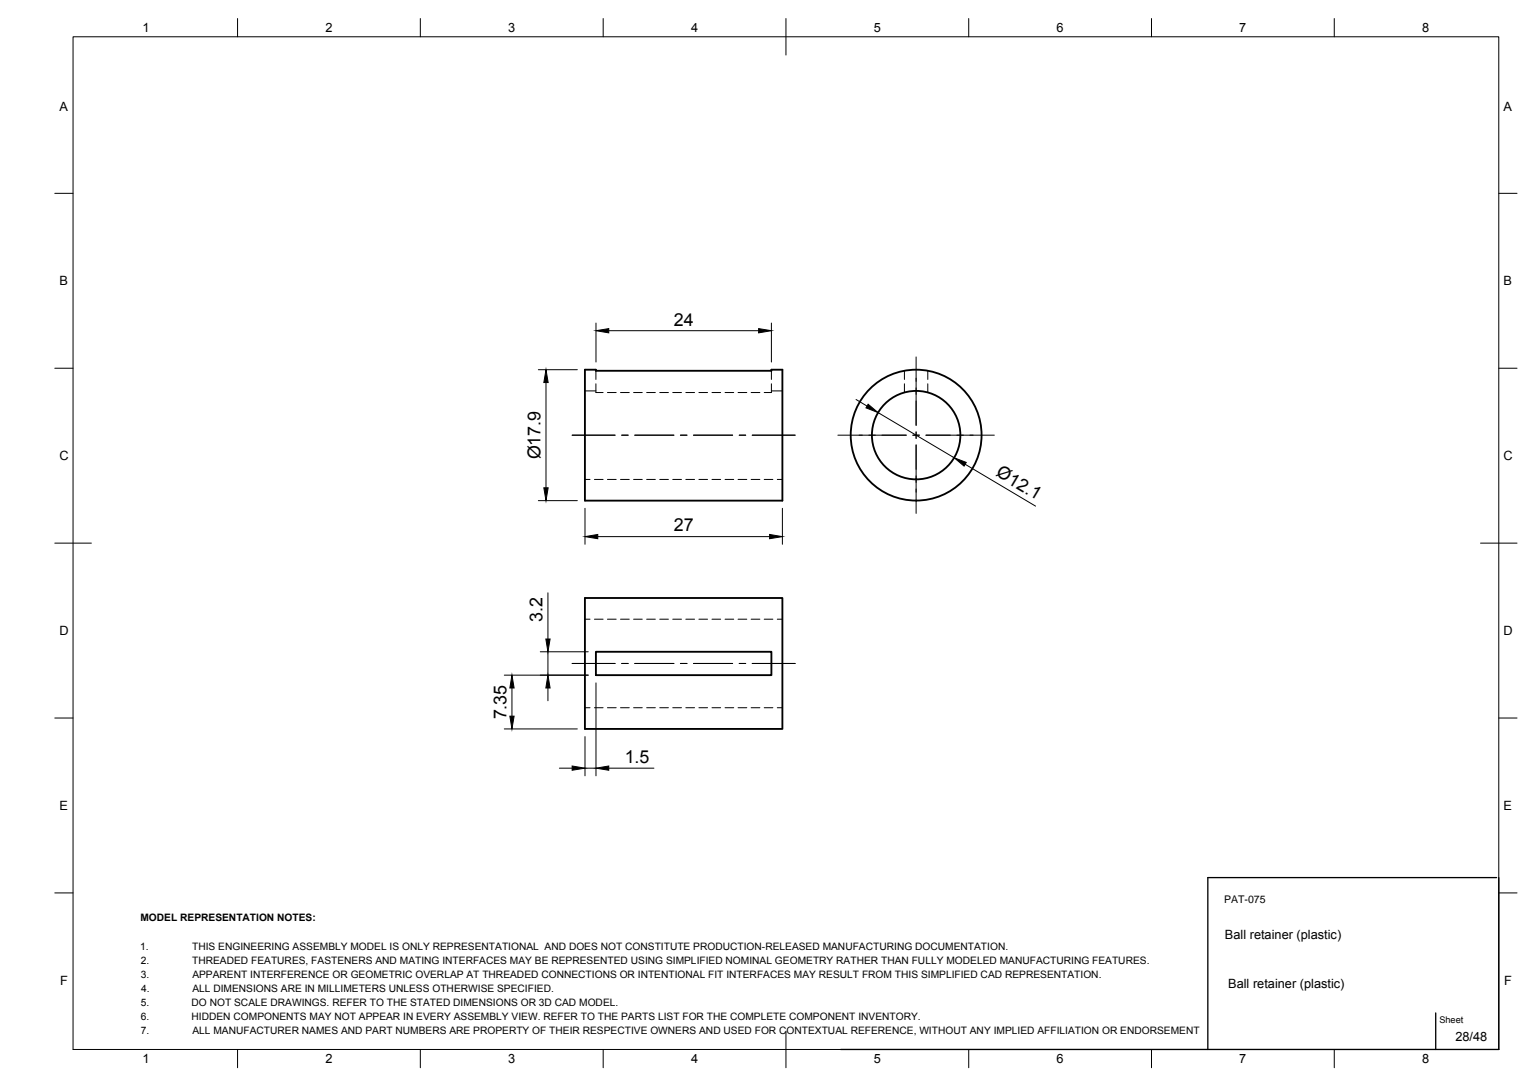
ISO-10303-21;
HEADER;
/* Generated by software containing ST-Developer
 * from STEP Tools, Inc. (www.steptools.com) 
 */

FILE_DESCRIPTION(
/* description */ ('Over-Centre Plunger Toggle Clamp on Slotted Fixture Frame'),
/* implementation_level */ '2;1');

FILE_NAME(
/* name */ 
'Ball retainer (plastic).step',
/* time_stamp */ '2026-10-28T03:23:24-07:00',
/* author */ (''),
/* organization */ (''),
/* preprocessor_version */ 'ST-DEVELOPER v20.2',
/* originating_system */ 'Autodesk Translation Framework v15.17.0.0',
/* authorisation */ '');

FILE_SCHEMA (('AUTOMOTIVE_DESIGN { 1 0 10303 214 3 1 1 }'));
ENDSEC;

DATA;
#10=MECHANICAL_DESIGN_GEOMETRIC_PRESENTATION_REPRESENTATION('',(#543),#15212);
#451=SHAPE_REPRESENTATION_RELATIONSHIP('SRR','None',#15427,#493);
#493=ADVANCED_BREP_SHAPE_REPRESENTATION('',(#593),#15189);
#543=STYLED_ITEM('',(#15712),#593);
#593=MANIFOLD_SOLID_BREP('Body1',#8276);
#736=FACE_BOUND('',#2002,.T.);
#737=FACE_BOUND('',#2004,.T.);
#738=FACE_BOUND('',#2006,.T.);
#739=FACE_BOUND('',#2008,.T.);
#966=PLANE('',#9332);
#967=PLANE('',#9335);
#968=PLANE('',#9336);
#969=PLANE('',#9339);
#970=PLANE('',#9340);
#971=PLANE('',#9345);
#1386=FACE_OUTER_BOUND('',#1997,.T.);
#1387=FACE_OUTER_BOUND('',#1998,.T.);
#1388=FACE_OUTER_BOUND('',#1999,.T.);
#1389=FACE_OUTER_BOUND('',#2000,.T.);
#1390=FACE_OUTER_BOUND('',#2001,.T.);
#1391=FACE_OUTER_BOUND('',#2003,.T.);
#1392=FACE_OUTER_BOUND('',#2005,.T.);
#1393=FACE_OUTER_BOUND('',#2007,.T.);
#1997=EDGE_LOOP('',(#6901,#6902,#6903,#6904));
#1998=EDGE_LOOP('',(#6905,#6906,#6907,#6908));
#1999=EDGE_LOOP('',(#6909,#6910,#6911,#6912));
#2000=EDGE_LOOP('',(#6913,#6914,#6915,#6916));
#2001=EDGE_LOOP('',(#6917));
#2002=EDGE_LOOP('',(#6918));
#2003=EDGE_LOOP('',(#6919,#6920,#6921,#6922));
#2004=EDGE_LOOP('',(#6923,#6924,#6925,#6926));
#2005=EDGE_LOOP('',(#6927));
#2006=EDGE_LOOP('',(#6928));
#2007=EDGE_LOOP('',(#6929,#6930,#6931,#6932));
#2008=EDGE_LOOP('',(#6933,#6934,#6935,#6936));
#2641=LINE('',#14158,#3271);
#2642=LINE('',#14161,#3272);
#2643=LINE('',#14164,#3273);
#2644=LINE('',#14166,#3274);
#2645=LINE('',#14167,#3275);
#2646=LINE('',#14173,#3276);
#2647=LINE('',#14175,#3277);
#2648=LINE('',#14176,#3278);
#2649=LINE('',#14185,#3279);
#2650=LINE('',#14190,#3280);
#3271=VECTOR('',#11306,1.);
#3272=VECTOR('',#11309,1.);
#3273=VECTOR('',#11312,1.);
#3274=VECTOR('',#11313,1.);
#3275=VECTOR('',#11314,1.);
#3276=VECTOR('',#11321,1.);
#3277=VECTOR('',#11324,1.);
#3278=VECTOR('',#11325,1.);
#3279=VECTOR('',#11336,0.895);
#3280=VECTOR('',#11343,0.605);
#3727=CIRCLE('',#9333,0.895);
#3728=CIRCLE('',#9334,0.605);
#3729=CIRCLE('',#9337,0.895);
#3730=CIRCLE('',#9338,0.605);
#3731=CIRCLE('',#9341,0.895);
#3732=CIRCLE('',#9342,0.605);
#3733=CIRCLE('',#9344,0.895);
#3734=CIRCLE('',#9346,0.605);
#4311=VERTEX_POINT('',#14154);
#4312=VERTEX_POINT('',#14155);
#4313=VERTEX_POINT('',#14157);
#4314=VERTEX_POINT('',#14159);
#4315=VERTEX_POINT('',#14163);
#4316=VERTEX_POINT('',#14165);
#4317=VERTEX_POINT('',#14169);
#4318=VERTEX_POINT('',#14171);
#4319=VERTEX_POINT('',#14178);
#4320=VERTEX_POINT('',#14180);
#4321=VERTEX_POINT('',#14183);
#4322=VERTEX_POINT('',#14187);
#5211=EDGE_CURVE('',#4311,#4312,#3727,.T.);
#5212=EDGE_CURVE('',#4313,#4311,#2641,.T.);
#5213=EDGE_CURVE('',#4314,#4313,#3728,.T.);
#5214=EDGE_CURVE('',#4312,#4314,#2642,.T.);
#5215=EDGE_CURVE('',#4312,#4315,#2643,.T.);
#5216=EDGE_CURVE('',#4316,#4314,#2644,.T.);
#5217=EDGE_CURVE('',#4316,#4315,#2645,.T.);
#5218=EDGE_CURVE('',#4315,#4317,#3729,.T.);
#5219=EDGE_CURVE('',#4318,#4316,#3730,.T.);
#5220=EDGE_CURVE('',#4317,#4318,#2646,.T.);
#5221=EDGE_CURVE('',#4317,#4311,#2647,.T.);
#5222=EDGE_CURVE('',#4313,#4318,#2648,.T.);
#5223=EDGE_CURVE('',#4319,#4319,#3731,.T.);
#5224=EDGE_CURVE('',#4320,#4320,#3732,.T.);
#5225=EDGE_CURVE('',#4321,#4321,#3733,.T.);
#5226=EDGE_CURVE('',#4321,#4319,#2649,.T.);
#5227=EDGE_CURVE('',#4322,#4322,#3734,.T.);
#5228=EDGE_CURVE('',#4322,#4320,#2650,.T.);
#6901=ORIENTED_EDGE('',*,*,#5211,.F.);
#6902=ORIENTED_EDGE('',*,*,#5212,.F.);
#6903=ORIENTED_EDGE('',*,*,#5213,.F.);
#6904=ORIENTED_EDGE('',*,*,#5214,.F.);
#6905=ORIENTED_EDGE('',*,*,#5215,.F.);
#6906=ORIENTED_EDGE('',*,*,#5214,.T.);
#6907=ORIENTED_EDGE('',*,*,#5216,.F.);
#6908=ORIENTED_EDGE('',*,*,#5217,.T.);
#6909=ORIENTED_EDGE('',*,*,#5218,.F.);
#6910=ORIENTED_EDGE('',*,*,#5217,.F.);
#6911=ORIENTED_EDGE('',*,*,#5219,.F.);
#6912=ORIENTED_EDGE('',*,*,#5220,.F.);
#6913=ORIENTED_EDGE('',*,*,#5221,.F.);
#6914=ORIENTED_EDGE('',*,*,#5220,.T.);
#6915=ORIENTED_EDGE('',*,*,#5222,.F.);
#6916=ORIENTED_EDGE('',*,*,#5212,.T.);
#6917=ORIENTED_EDGE('',*,*,#5223,.F.);
#6918=ORIENTED_EDGE('',*,*,#5224,.T.);
#6919=ORIENTED_EDGE('',*,*,#5225,.F.);
#6920=ORIENTED_EDGE('',*,*,#5226,.T.);
#6921=ORIENTED_EDGE('',*,*,#5223,.T.);
#6922=ORIENTED_EDGE('',*,*,#5226,.F.);
#6923=ORIENTED_EDGE('',*,*,#5218,.T.);
#6924=ORIENTED_EDGE('',*,*,#5221,.T.);
#6925=ORIENTED_EDGE('',*,*,#5211,.T.);
#6926=ORIENTED_EDGE('',*,*,#5215,.T.);
#6927=ORIENTED_EDGE('',*,*,#5225,.T.);
#6928=ORIENTED_EDGE('',*,*,#5227,.F.);
#6929=ORIENTED_EDGE('',*,*,#5227,.T.);
#6930=ORIENTED_EDGE('',*,*,#5228,.T.);
#6931=ORIENTED_EDGE('',*,*,#5224,.F.);
#6932=ORIENTED_EDGE('',*,*,#5228,.F.);
#6933=ORIENTED_EDGE('',*,*,#5219,.T.);
#6934=ORIENTED_EDGE('',*,*,#5216,.T.);
#6935=ORIENTED_EDGE('',*,*,#5213,.T.);
#6936=ORIENTED_EDGE('',*,*,#5222,.T.);
#7707=CYLINDRICAL_SURFACE('',#9343,0.895);
#7708=CYLINDRICAL_SURFACE('',#9347,0.605);
#8058=ADVANCED_FACE('',(#1386),#966,.F.);
#8059=ADVANCED_FACE('',(#1387),#967,.F.);
#8060=ADVANCED_FACE('',(#1388),#968,.F.);
#8061=ADVANCED_FACE('',(#1389),#969,.F.);
#8062=ADVANCED_FACE('',(#1390,#736),#970,.T.);
#8063=ADVANCED_FACE('',(#1391,#737),#7707,.T.);
#8064=ADVANCED_FACE('',(#1392,#738),#971,.T.);
#8065=ADVANCED_FACE('',(#1393,#739),#7708,.F.);
#8276=CLOSED_SHELL('',(#8058,#8059,#8060,#8061,#8062,#8063,#8064,#8065));
#9331=AXIS2_PLACEMENT_3D('',#14152,#11300,#11301);
#9332=AXIS2_PLACEMENT_3D('',#14153,#11302,#11303);
#9333=AXIS2_PLACEMENT_3D('',#14156,#11304,#11305);
#9334=AXIS2_PLACEMENT_3D('',#14160,#11307,#11308);
#9335=AXIS2_PLACEMENT_3D('',#14162,#11310,#11311);
#9336=AXIS2_PLACEMENT_3D('',#14168,#11315,#11316);
#9337=AXIS2_PLACEMENT_3D('',#14170,#11317,#11318);
#9338=AXIS2_PLACEMENT_3D('',#14172,#11319,#11320);
#9339=AXIS2_PLACEMENT_3D('',#14174,#11322,#11323);
#9340=AXIS2_PLACEMENT_3D('',#14177,#11326,#11327);
#9341=AXIS2_PLACEMENT_3D('',#14179,#11328,#11329);
#9342=AXIS2_PLACEMENT_3D('',#14181,#11330,#11331);
#9343=AXIS2_PLACEMENT_3D('',#14182,#11332,#11333);
#9344=AXIS2_PLACEMENT_3D('',#14184,#11334,#11335);
#9345=AXIS2_PLACEMENT_3D('',#14186,#11337,#11338);
#9346=AXIS2_PLACEMENT_3D('',#14188,#11339,#11340);
#9347=AXIS2_PLACEMENT_3D('',#14189,#11341,#11342);
#11300=DIRECTION('axis',(0.,0.,1.));
#11301=DIRECTION('refdir',(1.,0.,0.));
#11302=DIRECTION('center_axis',(0.,1.,0.));
#11303=DIRECTION('ref_axis',(0.,0.,1.));
#11304=DIRECTION('center_axis',(0.,1.,0.));
#11305=DIRECTION('ref_axis',(1.,0.,0.));
#11306=DIRECTION('',(1.,0.,0.));
#11307=DIRECTION('center_axis',(0.,-1.,0.));
#11308=DIRECTION('ref_axis',(1.,0.,0.));
#11309=DIRECTION('',(-1.,0.,0.));
#11310=DIRECTION('center_axis',(0.,0.,-1.));
#11311=DIRECTION('ref_axis',(-1.,0.,0.));
#11312=DIRECTION('',(0.,-1.,0.));
#11313=DIRECTION('',(0.,1.,0.));
#11314=DIRECTION('',(1.,0.,0.));
#11315=DIRECTION('center_axis',(0.,-1.,0.));
#11316=DIRECTION('ref_axis',(0.,0.,-1.));
#11317=DIRECTION('center_axis',(0.,-1.,0.));
#11318=DIRECTION('ref_axis',(1.,0.,0.));
#11319=DIRECTION('center_axis',(0.,1.,0.));
#11320=DIRECTION('ref_axis',(1.,0.,0.));
#11321=DIRECTION('',(-1.,0.,0.));
#11322=DIRECTION('center_axis',(0.,0.,1.));
#11323=DIRECTION('ref_axis',(1.,0.,0.));
#11324=DIRECTION('',(0.,1.,0.));
#11325=DIRECTION('',(0.,-1.,0.));
#11326=DIRECTION('center_axis',(0.,1.,0.));
#11327=DIRECTION('ref_axis',(0.,0.,1.));
#11328=DIRECTION('center_axis',(0.,-1.,0.));
#11329=DIRECTION('ref_axis',(1.,0.,0.));
#11330=DIRECTION('center_axis',(0.,-1.,0.));
#11331=DIRECTION('ref_axis',(1.,0.,0.));
#11332=DIRECTION('center_axis',(0.,-1.,0.));
#11333=DIRECTION('ref_axis',(1.,0.,0.));
#11334=DIRECTION('center_axis',(0.,-1.,0.));
#11335=DIRECTION('ref_axis',(1.,0.,0.));
#11336=DIRECTION('',(0.,1.,0.));
#11337=DIRECTION('center_axis',(0.,-1.,0.));
#11338=DIRECTION('ref_axis',(0.,0.,-1.));
#11339=DIRECTION('center_axis',(0.,-1.,0.));
#11340=DIRECTION('ref_axis',(1.,0.,0.));
#11341=DIRECTION('center_axis',(0.,-1.,0.));
#11342=DIRECTION('ref_axis',(1.,0.,0.));
#11343=DIRECTION('',(0.,1.,0.));
#14152=CARTESIAN_POINT('',(0.,0.,0.));
#14153=CARTESIAN_POINT('Origin',(0.75,1.2,0.));
#14154=CARTESIAN_POINT('',(0.880582193778639,1.2,0.16));
#14155=CARTESIAN_POINT('',(0.880582193778639,1.2,-0.16));
#14156=CARTESIAN_POINT('Origin',(0.,1.2,0.));
#14157=CARTESIAN_POINT('',(0.583459510163302,1.2,0.16));
#14158=CARTESIAN_POINT('',(0.57,1.2,0.16));
#14159=CARTESIAN_POINT('',(0.583459510163302,1.2,-0.16));
#14160=CARTESIAN_POINT('Origin',(0.,1.2,0.));
#14161=CARTESIAN_POINT('',(0.93,1.2,-0.16));
#14162=CARTESIAN_POINT('Origin',(0.93,0.,-0.16));
#14163=CARTESIAN_POINT('',(0.880582193778639,-1.2,-0.16));
#14164=CARTESIAN_POINT('',(0.880582193778639,0.,-0.16));
#14165=CARTESIAN_POINT('',(0.583459510163302,-1.2,-0.16));
#14166=CARTESIAN_POINT('',(0.583459510163302,0.,-0.16));
#14167=CARTESIAN_POINT('',(0.93,-1.2,-0.16));
#14168=CARTESIAN_POINT('Origin',(0.75,-1.2,0.));
#14169=CARTESIAN_POINT('',(0.880582193778639,-1.2,0.16));
#14170=CARTESIAN_POINT('Origin',(0.,-1.2,0.));
#14171=CARTESIAN_POINT('',(0.583459510163302,-1.2,0.16));
#14172=CARTESIAN_POINT('Origin',(0.,-1.2,0.));
#14173=CARTESIAN_POINT('',(0.57,-1.2,0.16));
#14174=CARTESIAN_POINT('Origin',(0.57,0.,0.16));
#14175=CARTESIAN_POINT('',(0.880582193778639,0.,0.16));
#14176=CARTESIAN_POINT('',(0.583459510163302,0.,0.16));
#14177=CARTESIAN_POINT('Origin',(0.895,1.35,0.));
#14178=CARTESIAN_POINT('',(-0.895,1.35,-1.09605888523688E-16));
#14179=CARTESIAN_POINT('Origin',(0.,1.35,0.));
#14180=CARTESIAN_POINT('',(-0.605,1.35,-7.40911313484149E-17));
#14181=CARTESIAN_POINT('Origin',(0.,1.35,0.));
#14182=CARTESIAN_POINT('Origin',(0.,0.,0.));
#14183=CARTESIAN_POINT('',(-0.895,-1.35,-1.09605888523688E-16));
#14184=CARTESIAN_POINT('Origin',(0.,-1.35,0.));
#14185=CARTESIAN_POINT('',(-0.895,0.,-1.09605888523688E-16));
#14186=CARTESIAN_POINT('Origin',(0.605,-1.35,0.));
#14187=CARTESIAN_POINT('',(-0.605,-1.35,-7.40911313484149E-17));
#14188=CARTESIAN_POINT('Origin',(0.,-1.35,0.));
#14189=CARTESIAN_POINT('Origin',(0.,0.,0.));
#14190=CARTESIAN_POINT('',(-0.605,0.,-7.40911313484149E-17));
#15139=UNCERTAINTY_MEASURE_WITH_UNIT(LENGTH_MEASURE(0.001),#15213,
'DISTANCE_ACCURACY_VALUE',
'Maximum model space distance between geometric entities at asserted c
onnectivities');
#15162=UNCERTAINTY_MEASURE_WITH_UNIT(LENGTH_MEASURE(0.001),#15213,
'DISTANCE_ACCURACY_VALUE',
'Maximum model space distance between geometric entities at asserted c
onnectivities');
#15189=(
GEOMETRIC_REPRESENTATION_CONTEXT(3)
GLOBAL_UNCERTAINTY_ASSIGNED_CONTEXT((#15139))
GLOBAL_UNIT_ASSIGNED_CONTEXT((#15213,#15215,#15216))
REPRESENTATION_CONTEXT('','3D')
);
#15212=(
GEOMETRIC_REPRESENTATION_CONTEXT(3)
GLOBAL_UNCERTAINTY_ASSIGNED_CONTEXT((#15162))
GLOBAL_UNIT_ASSIGNED_CONTEXT((#15213,#15215,#15216))
REPRESENTATION_CONTEXT('','3D')
);
#15213=(
LENGTH_UNIT()
NAMED_UNIT(*)
SI_UNIT(.CENTI.,.METRE.)
);
#15215=(
NAMED_UNIT(*)
PLANE_ANGLE_UNIT()
SI_UNIT($,.RADIAN.)
);
#15216=(
NAMED_UNIT(*)
SI_UNIT($,.STERADIAN.)
SOLID_ANGLE_UNIT()
);
#15243=SHAPE_DEFINITION_REPRESENTATION(#15297,#15427);
#15297=PRODUCT_DEFINITION_SHAPE('',$,#15477);
#15427=SHAPE_REPRESENTATION('',(#9331),#15189);
#15450=PRODUCT_DEFINITION_CONTEXT('part definition',#15599,'design');
#15477=PRODUCT_DEFINITION('Ball retainer (plastic)',
'Ball retainer (plastic)',#15526,#15450);
#15526=PRODUCT_DEFINITION_FORMATION('',$,#15627);
#15599=APPLICATION_CONTEXT(
'Core Data for Automotive Mechanical Design Process');
#15600=PRODUCT_CONTEXT('part definition',#15599,'mechanical');
#15627=PRODUCT('Ball retainer (plastic)','Ball retainer (plastic)',
'Ball retainer (plastic)',(#15600));
#15706=COLOUR_RGB('Sky Blue',0.24,0.69,0.87);
#15707=FILL_AREA_STYLE_COLOUR('',#15706);
#15708=FILL_AREA_STYLE('',(#15707));
#15709=SURFACE_STYLE_FILL_AREA(#15708);
#15710=SURFACE_SIDE_STYLE('',(#15709));
#15711=SURFACE_STYLE_USAGE(.BOTH.,#15710);
#15712=PRESENTATION_STYLE_ASSIGNMENT((#15711));
ENDSEC;
END-ISO-10303-21;
